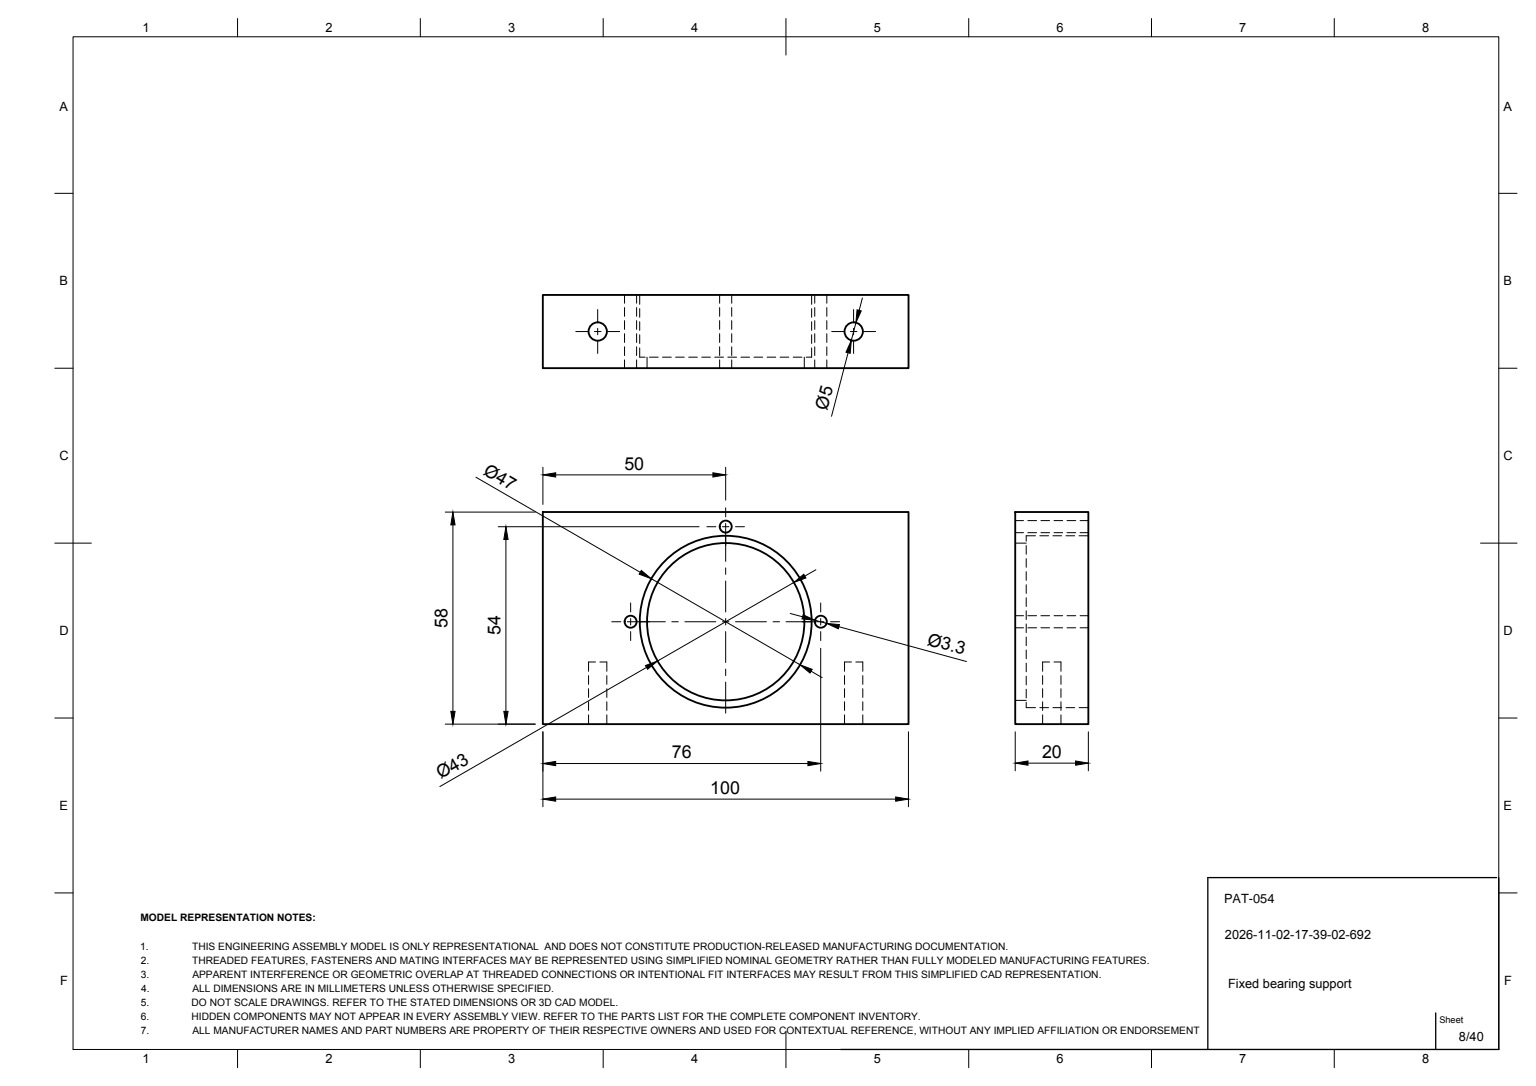
ISO-10303-21;
HEADER;
/* Generated by software containing ST-Developer
 * from STEP Tools, Inc. (www.steptools.com) 
 */

FILE_DESCRIPTION(
/* description */ ('PAT-054'),
/* implementation_level */ '2;1');

FILE_NAME(
/* name */ 'Fixed bearing support.step',
/* time_stamp */ '2026-10-29T16:38:13-07:00',
/* author */ (''),
/* organization */ (''),
/* preprocessor_version */ 'ST-DEVELOPER v20.2',
/* originating_system */ 'Autodesk Translation Framework v15.17.0.0',
/* authorisation */ '');

FILE_SCHEMA (('AUTOMOTIVE_DESIGN { 1 0 10303 214 3 1 1 }'));
ENDSEC;

DATA;
#10=MECHANICAL_DESIGN_GEOMETRIC_PRESENTATION_REPRESENTATION('',(#903),#33981);
#815=SHAPE_REPRESENTATION_RELATIONSHIP('SRR','None',#34188,#859);
#859=ADVANCED_BREP_SHAPE_REPRESENTATION('',(#962),#33936);
#903=STYLED_ITEM('',(#34517),#962);
#962=MANIFOLD_SOLID_BREP('Body1',#13014);
#1084=FACE_BOUND('',#2444,.T.);
#1085=FACE_BOUND('',#2452,.T.);
#1086=FACE_BOUND('',#2453,.T.);
#1087=FACE_BOUND('',#2454,.T.);
#1088=FACE_BOUND('',#2455,.T.);
#1089=FACE_BOUND('',#2458,.T.);
#1090=FACE_BOUND('',#2459,.T.);
#1091=FACE_BOUND('',#2460,.T.);
#1092=FACE_BOUND('',#2461,.T.);
#1093=FACE_BOUND('',#2464,.T.);
#1094=FACE_BOUND('',#2465,.T.);
#1256=PLANE('',#13729);
#1257=PLANE('',#13736);
#1258=PLANE('',#13740);
#1259=PLANE('',#13741);
#1260=PLANE('',#13742);
#1261=PLANE('',#13743);
#1262=PLANE('',#13744);
#1263=PLANE('',#13745);
#1264=PLANE('',#13746);
#1644=FACE_OUTER_BOUND('',#2439,.T.);
#1645=FACE_OUTER_BOUND('',#2440,.T.);
#1646=FACE_OUTER_BOUND('',#2441,.T.);
#1647=FACE_OUTER_BOUND('',#2442,.T.);
#1648=FACE_OUTER_BOUND('',#2443,.T.);
#1649=FACE_OUTER_BOUND('',#2445,.T.);
#1650=FACE_OUTER_BOUND('',#2446,.T.);
#1651=FACE_OUTER_BOUND('',#2447,.T.);
#1652=FACE_OUTER_BOUND('',#2448,.T.);
#1653=FACE_OUTER_BOUND('',#2449,.T.);
#1654=FACE_OUTER_BOUND('',#2450,.T.);
#1655=FACE_OUTER_BOUND('',#2451,.T.);
#1656=FACE_OUTER_BOUND('',#2456,.T.);
#1657=FACE_OUTER_BOUND('',#2457,.T.);
#1658=FACE_OUTER_BOUND('',#2462,.T.);
#1659=FACE_OUTER_BOUND('',#2463,.T.);
#2439=EDGE_LOOP('',(#8807,#8808,#8809,#8810));
#2440=EDGE_LOOP('',(#8811,#8812,#8813,#8814));
#2441=EDGE_LOOP('',(#8815,#8816,#8817,#8818));
#2442=EDGE_LOOP('',(#8819,#8820,#8821,#8822));
#2443=EDGE_LOOP('',(#8823));
#2444=EDGE_LOOP('',(#8824));
#2445=EDGE_LOOP('',(#8825,#8826,#8827,#8828));
#2446=EDGE_LOOP('',(#8829,#8830,#8831,#8832));
#2447=EDGE_LOOP('',(#8833));
#2448=EDGE_LOOP('',(#8834,#8835,#8836,#8837));
#2449=EDGE_LOOP('',(#8838));
#2450=EDGE_LOOP('',(#8839,#8840,#8841,#8842));
#2451=EDGE_LOOP('',(#8843,#8844,#8845,#8846));
#2452=EDGE_LOOP('',(#8847));
#2453=EDGE_LOOP('',(#8848));
#2454=EDGE_LOOP('',(#8849));
#2455=EDGE_LOOP('',(#8850));
#2456=EDGE_LOOP('',(#8851,#8852,#8853,#8854));
#2457=EDGE_LOOP('',(#8855,#8856,#8857,#8858));
#2458=EDGE_LOOP('',(#8859));
#2459=EDGE_LOOP('',(#8860));
#2460=EDGE_LOOP('',(#8861));
#2461=EDGE_LOOP('',(#8862));
#2462=EDGE_LOOP('',(#8863,#8864,#8865,#8866));
#2463=EDGE_LOOP('',(#8867,#8868,#8869,#8870));
#2464=EDGE_LOOP('',(#8871));
#2465=EDGE_LOOP('',(#8872));
#3314=LINE('',#18831,#4248);
#3315=LINE('',#18837,#4249);
#3316=LINE('',#18843,#4250);
#3317=LINE('',#18849,#4251);
#3318=LINE('',#18857,#4252);
#3319=LINE('',#18862,#4253);
#3320=LINE('',#18869,#4254);
#3321=LINE('',#18875,#4255);
#3322=LINE('',#18877,#4256);
#3323=LINE('',#18879,#4257);
#3324=LINE('',#18880,#4258);
#3325=LINE('',#18883,#4259);
#3326=LINE('',#18885,#4260);
#3327=LINE('',#18886,#4261);
#3328=LINE('',#18889,#4262);
#3329=LINE('',#18891,#4263);
#3330=LINE('',#18892,#4264);
#3331=LINE('',#18894,#4265);
#3332=LINE('',#18895,#4266);
#4248=VECTOR('',#15287,0.165);
#4249=VECTOR('',#15294,0.165);
#4250=VECTOR('',#15301,0.165);
#4251=VECTOR('',#15308,2.35);
#4252=VECTOR('',#15319,2.15);
#4253=VECTOR('',#15324,0.25);
#4254=VECTOR('',#15333,0.25);
#4255=VECTOR('',#15340,1.);
#4256=VECTOR('',#15341,1.);
#4257=VECTOR('',#15342,1.);
#4258=VECTOR('',#15343,1.);
#4259=VECTOR('',#15346,1.);
#4260=VECTOR('',#15347,1.);
#4261=VECTOR('',#15348,1.);
#4262=VECTOR('',#15351,1.);
#4263=VECTOR('',#15352,1.);
#4264=VECTOR('',#15353,1.);
#4265=VECTOR('',#15356,1.);
#4266=VECTOR('',#15357,1.);
#5187=CIRCLE('',#13718,0.165);
#5188=CIRCLE('',#13719,0.165);
#5189=CIRCLE('',#13721,0.165);
#5190=CIRCLE('',#13722,0.165);
#5191=CIRCLE('',#13724,0.165);
#5192=CIRCLE('',#13725,0.165);
#5193=CIRCLE('',#13727,2.35);
#5194=CIRCLE('',#13728,2.35);
#5195=CIRCLE('',#13730,2.15);
#5196=CIRCLE('',#13732,2.15);
#5197=CIRCLE('',#13734,0.25);
#5198=CIRCLE('',#13735,0.25);
#5199=CIRCLE('',#13738,0.25);
#5200=CIRCLE('',#13739,0.25);
#5676=VERTEX_POINT('',#18828);
#5677=VERTEX_POINT('',#18830);
#5678=VERTEX_POINT('',#18834);
#5679=VERTEX_POINT('',#18836);
#5680=VERTEX_POINT('',#18840);
#5681=VERTEX_POINT('',#18842);
#5682=VERTEX_POINT('',#18846);
#5683=VERTEX_POINT('',#18848);
#5684=VERTEX_POINT('',#18852);
#5685=VERTEX_POINT('',#18855);
#5686=VERTEX_POINT('',#18859);
#5687=VERTEX_POINT('',#18861);
#5688=VERTEX_POINT('',#18866);
#5689=VERTEX_POINT('',#18868);
#5690=VERTEX_POINT('',#18873);
#5691=VERTEX_POINT('',#18874);
#5692=VERTEX_POINT('',#18876);
#5693=VERTEX_POINT('',#18878);
#5694=VERTEX_POINT('',#18882);
#5695=VERTEX_POINT('',#18884);
#5696=VERTEX_POINT('',#18888);
#5697=VERTEX_POINT('',#18890);
#6903=EDGE_CURVE('',#5676,#5676,#5187,.T.);
#6904=EDGE_CURVE('',#5676,#5677,#3314,.T.);
#6905=EDGE_CURVE('',#5677,#5677,#5188,.T.);
#6906=EDGE_CURVE('',#5678,#5678,#5189,.T.);
#6907=EDGE_CURVE('',#5678,#5679,#3315,.T.);
#6908=EDGE_CURVE('',#5679,#5679,#5190,.T.);
#6909=EDGE_CURVE('',#5680,#5680,#5191,.T.);
#6910=EDGE_CURVE('',#5680,#5681,#3316,.T.);
#6911=EDGE_CURVE('',#5681,#5681,#5192,.T.);
#6912=EDGE_CURVE('',#5682,#5682,#5193,.T.);
#6913=EDGE_CURVE('',#5682,#5683,#3317,.T.);
#6914=EDGE_CURVE('',#5683,#5683,#5194,.T.);
#6915=EDGE_CURVE('',#5684,#5684,#5195,.T.);
#6916=EDGE_CURVE('',#5685,#5685,#5196,.T.);
#6917=EDGE_CURVE('',#5685,#5684,#3318,.T.);
#6918=EDGE_CURVE('',#5686,#5686,#5197,.T.);
#6919=EDGE_CURVE('',#5686,#5687,#3319,.T.);
#6920=EDGE_CURVE('',#5687,#5687,#5198,.T.);
#6921=EDGE_CURVE('',#5688,#5688,#5199,.T.);
#6922=EDGE_CURVE('',#5688,#5689,#3320,.T.);
#6923=EDGE_CURVE('',#5689,#5689,#5200,.T.);
#6924=EDGE_CURVE('',#5690,#5691,#3321,.T.);
#6925=EDGE_CURVE('',#5691,#5692,#3322,.T.);
#6926=EDGE_CURVE('',#5693,#5692,#3323,.T.);
#6927=EDGE_CURVE('',#5690,#5693,#3324,.T.);
#6928=EDGE_CURVE('',#5694,#5690,#3325,.T.);
#6929=EDGE_CURVE('',#5695,#5693,#3326,.T.);
#6930=EDGE_CURVE('',#5694,#5695,#3327,.T.);
#6931=EDGE_CURVE('',#5696,#5694,#3328,.T.);
#6932=EDGE_CURVE('',#5697,#5695,#3329,.T.);
#6933=EDGE_CURVE('',#5696,#5697,#3330,.T.);
#6934=EDGE_CURVE('',#5691,#5696,#3331,.T.);
#6935=EDGE_CURVE('',#5692,#5697,#3332,.T.);
#8807=ORIENTED_EDGE('',*,*,#6903,.F.);
#8808=ORIENTED_EDGE('',*,*,#6904,.T.);
#8809=ORIENTED_EDGE('',*,*,#6905,.F.);
#8810=ORIENTED_EDGE('',*,*,#6904,.F.);
#8811=ORIENTED_EDGE('',*,*,#6906,.F.);
#8812=ORIENTED_EDGE('',*,*,#6907,.T.);
#8813=ORIENTED_EDGE('',*,*,#6908,.F.);
#8814=ORIENTED_EDGE('',*,*,#6907,.F.);
#8815=ORIENTED_EDGE('',*,*,#6909,.F.);
#8816=ORIENTED_EDGE('',*,*,#6910,.T.);
#8817=ORIENTED_EDGE('',*,*,#6911,.F.);
#8818=ORIENTED_EDGE('',*,*,#6910,.F.);
#8819=ORIENTED_EDGE('',*,*,#6912,.F.);
#8820=ORIENTED_EDGE('',*,*,#6913,.T.);
#8821=ORIENTED_EDGE('',*,*,#6914,.F.);
#8822=ORIENTED_EDGE('',*,*,#6913,.F.);
#8823=ORIENTED_EDGE('',*,*,#6912,.T.);
#8824=ORIENTED_EDGE('',*,*,#6915,.F.);
#8825=ORIENTED_EDGE('',*,*,#6916,.F.);
#8826=ORIENTED_EDGE('',*,*,#6917,.T.);
#8827=ORIENTED_EDGE('',*,*,#6915,.T.);
#8828=ORIENTED_EDGE('',*,*,#6917,.F.);
#8829=ORIENTED_EDGE('',*,*,#6918,.F.);
#8830=ORIENTED_EDGE('',*,*,#6919,.T.);
#8831=ORIENTED_EDGE('',*,*,#6920,.T.);
#8832=ORIENTED_EDGE('',*,*,#6919,.F.);
#8833=ORIENTED_EDGE('',*,*,#6920,.F.);
#8834=ORIENTED_EDGE('',*,*,#6921,.F.);
#8835=ORIENTED_EDGE('',*,*,#6922,.T.);
#8836=ORIENTED_EDGE('',*,*,#6923,.T.);
#8837=ORIENTED_EDGE('',*,*,#6922,.F.);
#8838=ORIENTED_EDGE('',*,*,#6923,.F.);
#8839=ORIENTED_EDGE('',*,*,#6924,.T.);
#8840=ORIENTED_EDGE('',*,*,#6925,.T.);
#8841=ORIENTED_EDGE('',*,*,#6926,.F.);
#8842=ORIENTED_EDGE('',*,*,#6927,.F.);
#8843=ORIENTED_EDGE('',*,*,#6928,.T.);
#8844=ORIENTED_EDGE('',*,*,#6927,.T.);
#8845=ORIENTED_EDGE('',*,*,#6929,.F.);
#8846=ORIENTED_EDGE('',*,*,#6930,.F.);
#8847=ORIENTED_EDGE('',*,*,#6905,.T.);
#8848=ORIENTED_EDGE('',*,*,#6908,.T.);
#8849=ORIENTED_EDGE('',*,*,#6911,.T.);
#8850=ORIENTED_EDGE('',*,*,#6914,.T.);
#8851=ORIENTED_EDGE('',*,*,#6931,.T.);
#8852=ORIENTED_EDGE('',*,*,#6930,.T.);
#8853=ORIENTED_EDGE('',*,*,#6932,.F.);
#8854=ORIENTED_EDGE('',*,*,#6933,.F.);
#8855=ORIENTED_EDGE('',*,*,#6934,.T.);
#8856=ORIENTED_EDGE('',*,*,#6933,.T.);
#8857=ORIENTED_EDGE('',*,*,#6935,.F.);
#8858=ORIENTED_EDGE('',*,*,#6925,.F.);
#8859=ORIENTED_EDGE('',*,*,#6903,.T.);
#8860=ORIENTED_EDGE('',*,*,#6906,.T.);
#8861=ORIENTED_EDGE('',*,*,#6909,.T.);
#8862=ORIENTED_EDGE('',*,*,#6916,.T.);
#8863=ORIENTED_EDGE('',*,*,#6935,.T.);
#8864=ORIENTED_EDGE('',*,*,#6932,.T.);
#8865=ORIENTED_EDGE('',*,*,#6929,.T.);
#8866=ORIENTED_EDGE('',*,*,#6926,.T.);
#8867=ORIENTED_EDGE('',*,*,#6934,.F.);
#8868=ORIENTED_EDGE('',*,*,#6924,.F.);
#8869=ORIENTED_EDGE('',*,*,#6928,.F.);
#8870=ORIENTED_EDGE('',*,*,#6931,.F.);
#8871=ORIENTED_EDGE('',*,*,#6918,.T.);
#8872=ORIENTED_EDGE('',*,*,#6921,.T.);
#12020=CYLINDRICAL_SURFACE('',#13717,0.165);
#12021=CYLINDRICAL_SURFACE('',#13720,0.165);
#12022=CYLINDRICAL_SURFACE('',#13723,0.165);
#12023=CYLINDRICAL_SURFACE('',#13726,2.35);
#12024=CYLINDRICAL_SURFACE('',#13731,2.15);
#12025=CYLINDRICAL_SURFACE('',#13733,0.25);
#12026=CYLINDRICAL_SURFACE('',#13737,0.25);
#12356=ADVANCED_FACE('',(#1644),#12020,.F.);
#12357=ADVANCED_FACE('',(#1645),#12021,.F.);
#12358=ADVANCED_FACE('',(#1646),#12022,.F.);
#12359=ADVANCED_FACE('',(#1647),#12023,.F.);
#12360=ADVANCED_FACE('',(#1648,#1084),#1256,.T.);
#12361=ADVANCED_FACE('',(#1649),#12024,.F.);
#12362=ADVANCED_FACE('',(#1650),#12025,.F.);
#12363=ADVANCED_FACE('',(#1651),#1257,.F.);
#12364=ADVANCED_FACE('',(#1652),#12026,.F.);
#12365=ADVANCED_FACE('',(#1653),#1258,.F.);
#12366=ADVANCED_FACE('',(#1654),#1259,.T.);
#12367=ADVANCED_FACE('',(#1655,#1085,#1086,#1087,#1088),#1260,.T.);
#12368=ADVANCED_FACE('',(#1656),#1261,.T.);
#12369=ADVANCED_FACE('',(#1657,#1089,#1090,#1091,#1092),#1262,.T.);
#12370=ADVANCED_FACE('',(#1658),#1263,.T.);
#12371=ADVANCED_FACE('',(#1659,#1093,#1094),#1264,.F.);
#13014=CLOSED_SHELL('',(#12356,#12357,#12358,#12359,#12360,#12361,#12362,
#12363,#12364,#12365,#12366,#12367,#12368,#12369,#12370,#12371));
#13716=AXIS2_PLACEMENT_3D('',#18826,#15281,#15282);
#13717=AXIS2_PLACEMENT_3D('',#18827,#15283,#15284);
#13718=AXIS2_PLACEMENT_3D('',#18829,#15285,#15286);
#13719=AXIS2_PLACEMENT_3D('',#18832,#15288,#15289);
#13720=AXIS2_PLACEMENT_3D('',#18833,#15290,#15291);
#13721=AXIS2_PLACEMENT_3D('',#18835,#15292,#15293);
#13722=AXIS2_PLACEMENT_3D('',#18838,#15295,#15296);
#13723=AXIS2_PLACEMENT_3D('',#18839,#15297,#15298);
#13724=AXIS2_PLACEMENT_3D('',#18841,#15299,#15300);
#13725=AXIS2_PLACEMENT_3D('',#18844,#15302,#15303);
#13726=AXIS2_PLACEMENT_3D('',#18845,#15304,#15305);
#13727=AXIS2_PLACEMENT_3D('',#18847,#15306,#15307);
#13728=AXIS2_PLACEMENT_3D('',#18850,#15309,#15310);
#13729=AXIS2_PLACEMENT_3D('',#18851,#15311,#15312);
#13730=AXIS2_PLACEMENT_3D('',#18853,#15313,#15314);
#13731=AXIS2_PLACEMENT_3D('',#18854,#15315,#15316);
#13732=AXIS2_PLACEMENT_3D('',#18856,#15317,#15318);
#13733=AXIS2_PLACEMENT_3D('',#18858,#15320,#15321);
#13734=AXIS2_PLACEMENT_3D('',#18860,#15322,#15323);
#13735=AXIS2_PLACEMENT_3D('',#18863,#15325,#15326);
#13736=AXIS2_PLACEMENT_3D('',#18864,#15327,#15328);
#13737=AXIS2_PLACEMENT_3D('',#18865,#15329,#15330);
#13738=AXIS2_PLACEMENT_3D('',#18867,#15331,#15332);
#13739=AXIS2_PLACEMENT_3D('',#18870,#15334,#15335);
#13740=AXIS2_PLACEMENT_3D('',#18871,#15336,#15337);
#13741=AXIS2_PLACEMENT_3D('',#18872,#15338,#15339);
#13742=AXIS2_PLACEMENT_3D('',#18881,#15344,#15345);
#13743=AXIS2_PLACEMENT_3D('',#18887,#15349,#15350);
#13744=AXIS2_PLACEMENT_3D('',#18893,#15354,#15355);
#13745=AXIS2_PLACEMENT_3D('',#18896,#15358,#15359);
#13746=AXIS2_PLACEMENT_3D('',#18897,#15360,#15361);
#15281=DIRECTION('axis',(0.,0.,1.));
#15282=DIRECTION('refdir',(1.,0.,0.));
#15283=DIRECTION('center_axis',(1.,0.,0.));
#15284=DIRECTION('ref_axis',(0.,0.,-1.));
#15285=DIRECTION('center_axis',(1.,0.,0.));
#15286=DIRECTION('ref_axis',(0.,0.,-1.));
#15287=DIRECTION('',(1.,0.,0.));
#15288=DIRECTION('center_axis',(-1.,0.,0.));
#15289=DIRECTION('ref_axis',(0.,0.,-1.));
#15290=DIRECTION('center_axis',(1.,0.,0.));
#15291=DIRECTION('ref_axis',(0.,0.,-1.));
#15292=DIRECTION('center_axis',(1.,0.,0.));
#15293=DIRECTION('ref_axis',(0.,0.,-1.));
#15294=DIRECTION('',(1.,0.,0.));
#15295=DIRECTION('center_axis',(-1.,0.,0.));
#15296=DIRECTION('ref_axis',(0.,0.,-1.));
#15297=DIRECTION('center_axis',(1.,0.,0.));
#15298=DIRECTION('ref_axis',(0.,0.,-1.));
#15299=DIRECTION('center_axis',(1.,0.,0.));
#15300=DIRECTION('ref_axis',(0.,0.,-1.));
#15301=DIRECTION('',(1.,0.,0.));
#15302=DIRECTION('center_axis',(-1.,0.,0.));
#15303=DIRECTION('ref_axis',(0.,0.,-1.));
#15304=DIRECTION('center_axis',(1.,0.,0.));
#15305=DIRECTION('ref_axis',(0.,0.,-1.));
#15306=DIRECTION('center_axis',(1.,0.,0.));
#15307=DIRECTION('ref_axis',(0.,0.,-1.));
#15308=DIRECTION('',(1.,0.,0.));
#15309=DIRECTION('center_axis',(-1.,0.,0.));
#15310=DIRECTION('ref_axis',(0.,0.,-1.));
#15311=DIRECTION('center_axis',(1.,0.,0.));
#15312=DIRECTION('ref_axis',(0.,0.,-1.));
#15313=DIRECTION('center_axis',(1.,0.,0.));
#15314=DIRECTION('ref_axis',(0.,0.,-1.));
#15315=DIRECTION('center_axis',(1.,0.,0.));
#15316=DIRECTION('ref_axis',(0.,0.,-1.));
#15317=DIRECTION('center_axis',(1.,0.,0.));
#15318=DIRECTION('ref_axis',(0.,0.,-1.));
#15319=DIRECTION('',(1.,0.,0.));
#15320=DIRECTION('center_axis',(0.,0.,1.));
#15321=DIRECTION('ref_axis',(1.,0.,0.));
#15322=DIRECTION('center_axis',(0.,0.,1.));
#15323=DIRECTION('ref_axis',(1.,0.,0.));
#15324=DIRECTION('',(0.,0.,1.));
#15325=DIRECTION('center_axis',(0.,0.,1.));
#15326=DIRECTION('ref_axis',(1.,0.,0.));
#15327=DIRECTION('center_axis',(0.,0.,1.));
#15328=DIRECTION('ref_axis',(1.,0.,0.));
#15329=DIRECTION('center_axis',(0.,0.,1.));
#15330=DIRECTION('ref_axis',(1.,0.,0.));
#15331=DIRECTION('center_axis',(0.,0.,1.));
#15332=DIRECTION('ref_axis',(1.,0.,0.));
#15333=DIRECTION('',(0.,0.,1.));
#15334=DIRECTION('center_axis',(0.,0.,1.));
#15335=DIRECTION('ref_axis',(1.,0.,0.));
#15336=DIRECTION('center_axis',(0.,0.,1.));
#15337=DIRECTION('ref_axis',(1.,0.,0.));
#15338=DIRECTION('center_axis',(0.,1.,0.));
#15339=DIRECTION('ref_axis',(-1.,0.,0.));
#15340=DIRECTION('',(-1.,0.,0.));
#15341=DIRECTION('',(0.,0.,1.));
#15342=DIRECTION('',(-1.,0.,0.));
#15343=DIRECTION('',(0.,0.,1.));
#15344=DIRECTION('center_axis',(1.,0.,0.));
#15345=DIRECTION('ref_axis',(0.,1.,0.));
#15346=DIRECTION('',(0.,1.,0.));
#15347=DIRECTION('',(0.,1.,0.));
#15348=DIRECTION('',(0.,0.,1.));
#15349=DIRECTION('center_axis',(0.,-1.,0.));
#15350=DIRECTION('ref_axis',(1.,0.,0.));
#15351=DIRECTION('',(1.,0.,0.));
#15352=DIRECTION('',(1.,0.,0.));
#15353=DIRECTION('',(0.,0.,1.));
#15354=DIRECTION('center_axis',(-1.,0.,0.));
#15355=DIRECTION('ref_axis',(0.,-1.,0.));
#15356=DIRECTION('',(0.,-1.,0.));
#15357=DIRECTION('',(0.,-1.,0.));
#15358=DIRECTION('center_axis',(0.,0.,1.));
#15359=DIRECTION('ref_axis',(1.,0.,0.));
#15360=DIRECTION('center_axis',(0.,0.,1.));
#15361=DIRECTION('ref_axis',(1.,0.,0.));
#18826=CARTESIAN_POINT('',(0.,0.,0.));
#18827=CARTESIAN_POINT('Origin',(22.9,-2.6,4.));
#18828=CARTESIAN_POINT('',(23.,-2.6,4.165));
#18829=CARTESIAN_POINT('Origin',(23.,-2.6,4.));
#18830=CARTESIAN_POINT('',(25.,-2.6,4.165));
#18831=CARTESIAN_POINT('',(22.9,-2.6,4.165));
#18832=CARTESIAN_POINT('Origin',(25.,-2.6,4.));
#18833=CARTESIAN_POINT('Origin',(22.9,2.6,4.));
#18834=CARTESIAN_POINT('',(23.,2.6,4.165));
#18835=CARTESIAN_POINT('Origin',(23.,2.6,4.));
#18836=CARTESIAN_POINT('',(25.,2.6,4.165));
#18837=CARTESIAN_POINT('',(22.9,2.6,4.165));
#18838=CARTESIAN_POINT('Origin',(25.,2.6,4.));
#18839=CARTESIAN_POINT('Origin',(22.9,0.,6.6));
#18840=CARTESIAN_POINT('',(23.,-2.02066721859313E-17,6.765));
#18841=CARTESIAN_POINT('Origin',(23.,0.,6.6));
#18842=CARTESIAN_POINT('',(25.,2.02066721859313E-17,6.765));
#18843=CARTESIAN_POINT('',(22.9,-2.02066721859313E-17,6.765));
#18844=CARTESIAN_POINT('Origin',(25.,0.,6.6));
#18845=CARTESIAN_POINT('Origin',(23.3,0.,4.));
#18846=CARTESIAN_POINT('',(23.3,-2.87791997799628E-16,6.35));
#18847=CARTESIAN_POINT('Origin',(23.3,0.,4.));
#18848=CARTESIAN_POINT('',(25.,2.87791997799628E-16,6.35));
#18849=CARTESIAN_POINT('',(23.3,-2.87791997799628E-16,6.35));
#18850=CARTESIAN_POINT('Origin',(25.,0.,4.));
#18851=CARTESIAN_POINT('Origin',(23.3,0.,4.));
#18852=CARTESIAN_POINT('',(23.3,-2.63299061816681E-16,6.15));
#18853=CARTESIAN_POINT('Origin',(23.3,0.,4.));
#18854=CARTESIAN_POINT('Origin',(22.9,0.,4.));
#18855=CARTESIAN_POINT('',(23.,-2.63299061816681E-16,6.15));
#18856=CARTESIAN_POINT('Origin',(23.,0.,4.));
#18857=CARTESIAN_POINT('',(22.9,-2.63299061816681E-16,6.15));
#18858=CARTESIAN_POINT('Origin',(24.,-3.5,1.1));
#18859=CARTESIAN_POINT('',(23.75,-3.5,1.2));
#18860=CARTESIAN_POINT('Origin',(24.,-3.5,1.2));
#18861=CARTESIAN_POINT('',(23.75,-3.5,2.9));
#18862=CARTESIAN_POINT('',(23.75,-3.5,1.1));
#18863=CARTESIAN_POINT('Origin',(24.,-3.5,2.9));
#18864=CARTESIAN_POINT('Origin',(24.,-3.5,2.9));
#18865=CARTESIAN_POINT('Origin',(24.,3.5,1.1));
#18866=CARTESIAN_POINT('',(23.75,3.5,1.2));
#18867=CARTESIAN_POINT('Origin',(24.,3.5,1.2));
#18868=CARTESIAN_POINT('',(23.75,3.5,2.9));
#18869=CARTESIAN_POINT('',(23.75,3.5,1.1));
#18870=CARTESIAN_POINT('Origin',(24.,3.5,2.9));
#18871=CARTESIAN_POINT('Origin',(24.,3.5,2.9));
#18872=CARTESIAN_POINT('Origin',(25.,5.,1.2));
#18873=CARTESIAN_POINT('',(25.,5.,1.2));
#18874=CARTESIAN_POINT('',(23.,5.,1.2));
#18875=CARTESIAN_POINT('',(25.,5.,1.2));
#18876=CARTESIAN_POINT('',(23.,5.,7.));
#18877=CARTESIAN_POINT('',(23.,5.,1.2));
#18878=CARTESIAN_POINT('',(25.,5.,7.));
#18879=CARTESIAN_POINT('',(25.,5.,7.));
#18880=CARTESIAN_POINT('',(25.,5.,1.2));
#18881=CARTESIAN_POINT('Origin',(25.,-5.,1.2));
#18882=CARTESIAN_POINT('',(25.,-5.,1.2));
#18883=CARTESIAN_POINT('',(25.,-5.,1.2));
#18884=CARTESIAN_POINT('',(25.,-5.,7.));
#18885=CARTESIAN_POINT('',(25.,-5.,7.));
#18886=CARTESIAN_POINT('',(25.,-5.,1.2));
#18887=CARTESIAN_POINT('Origin',(23.,-5.,1.2));
#18888=CARTESIAN_POINT('',(23.,-5.,1.2));
#18889=CARTESIAN_POINT('',(23.,-5.,1.2));
#18890=CARTESIAN_POINT('',(23.,-5.,7.));
#18891=CARTESIAN_POINT('',(23.,-5.,7.));
#18892=CARTESIAN_POINT('',(23.,-5.,1.2));
#18893=CARTESIAN_POINT('Origin',(23.,5.,1.2));
#18894=CARTESIAN_POINT('',(23.,5.,1.2));
#18895=CARTESIAN_POINT('',(23.,5.,7.));
#18896=CARTESIAN_POINT('Origin',(24.,0.,7.));
#18897=CARTESIAN_POINT('Origin',(24.,0.,1.2));
#33884=UNCERTAINTY_MEASURE_WITH_UNIT(LENGTH_MEASURE(0.001),#33982,
'DISTANCE_ACCURACY_VALUE',
'Maximum model space distance between geometric entities at asserted c
onnectivities');
#33929=UNCERTAINTY_MEASURE_WITH_UNIT(LENGTH_MEASURE(0.001),#33982,
'DISTANCE_ACCURACY_VALUE',
'Maximum model space distance between geometric entities at asserted c
onnectivities');
#33936=(
GEOMETRIC_REPRESENTATION_CONTEXT(3)
GLOBAL_UNCERTAINTY_ASSIGNED_CONTEXT((#33884))
GLOBAL_UNIT_ASSIGNED_CONTEXT((#33982,#33984,#33985))
REPRESENTATION_CONTEXT('','3D')
);
#33981=(
GEOMETRIC_REPRESENTATION_CONTEXT(3)
GLOBAL_UNCERTAINTY_ASSIGNED_CONTEXT((#33929))
GLOBAL_UNIT_ASSIGNED_CONTEXT((#33982,#33984,#33985))
REPRESENTATION_CONTEXT('','3D')
);
#33982=(
LENGTH_UNIT()
NAMED_UNIT(*)
SI_UNIT(.CENTI.,.METRE.)
);
#33984=(
NAMED_UNIT(*)
PLANE_ANGLE_UNIT()
SI_UNIT($,.RADIAN.)
);
#33985=(
NAMED_UNIT(*)
SI_UNIT($,.STERADIAN.)
SOLID_ANGLE_UNIT()
);
#33992=SHAPE_DEFINITION_REPRESENTATION(#34043,#34188);
#34043=PRODUCT_DEFINITION_SHAPE('',$,#34240);
#34188=SHAPE_REPRESENTATION('',(#13716),#33936);
#34233=PRODUCT_DEFINITION_CONTEXT('part definition',#34388,'design');
#34240=PRODUCT_DEFINITION('Fixed bearing support',
'Fixed bearing support',#34291,#34233);
#34291=PRODUCT_DEFINITION_FORMATION('',$,#34396);
#34388=APPLICATION_CONTEXT(
'Core Data for Automotive Mechanical Design Process');
#34389=PRODUCT_CONTEXT('part definition',#34388,'mechanical');
#34396=PRODUCT('Fixed bearing support','Fixed bearing support',
'Fixed bearing support',(#34389));
#34511=COLOUR_RGB('Grey',0.48,0.52,0.57);
#34512=FILL_AREA_STYLE_COLOUR('',#34511);
#34513=FILL_AREA_STYLE('',(#34512));
#34514=SURFACE_STYLE_FILL_AREA(#34513);
#34515=SURFACE_SIDE_STYLE('',(#34514));
#34516=SURFACE_STYLE_USAGE(.BOTH.,#34515);
#34517=PRESENTATION_STYLE_ASSIGNMENT((#34516));
ENDSEC;
END-ISO-10303-21;
